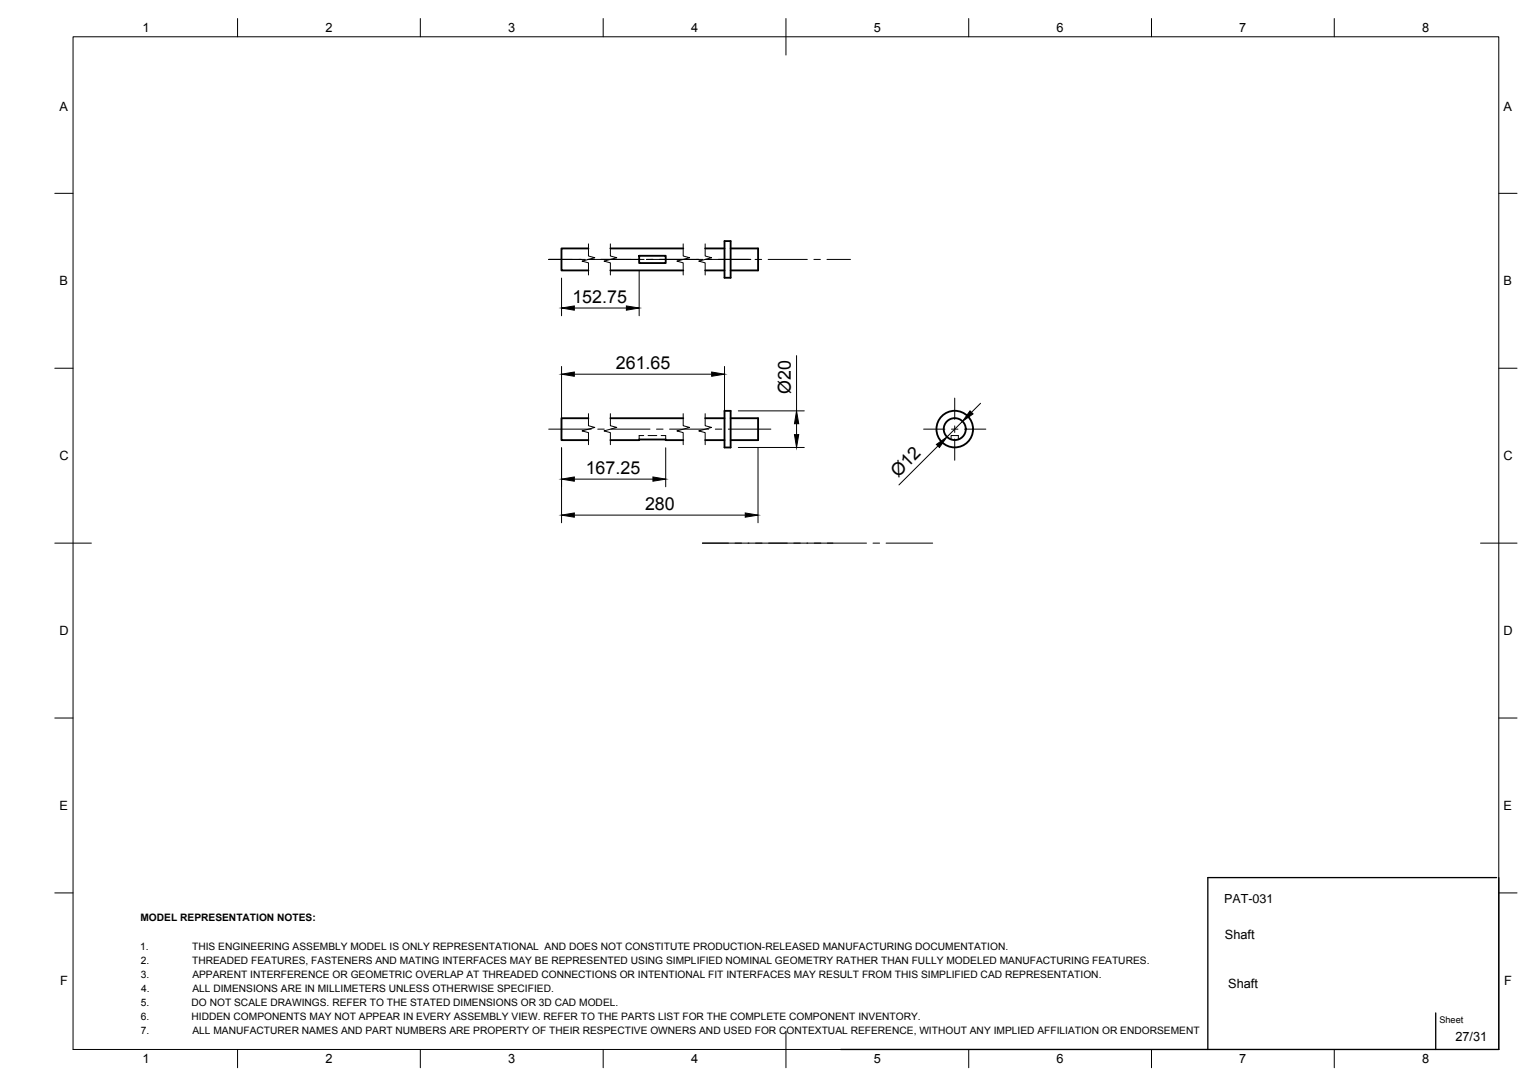
ISO-10303-21;
HEADER;
/* Generated by software containing ST-Developer
 * from STEP Tools, Inc. (www.steptools.com) 
 */

FILE_DESCRIPTION(
/* description */ ('Double-row support with tensioned shaft'),
/* implementation_level */ '2;1');

FILE_NAME(
/* name */ 'Shaft.step',
/* time_stamp */ '2026-10-27T10:50:35-07:00',
/* author */ (''),
/* organization */ (''),
/* preprocessor_version */ 'ST-DEVELOPER v20.2',
/* originating_system */ 'Autodesk Translation Framework v15.17.0.0',
/* authorisation */ '');

FILE_SCHEMA (('AUTOMOTIVE_DESIGN { 1 0 10303 214 3 1 1 }'));
ENDSEC;

DATA;
#10=MECHANICAL_DESIGN_GEOMETRIC_PRESENTATION_REPRESENTATION('',(#504),#11559);
#439=SHAPE_REPRESENTATION_RELATIONSHIP('SRR','None',#11749,#471);
#471=ADVANCED_BREP_SHAPE_REPRESENTATION('',(#534),#11551);
#504=STYLED_ITEM('',(#11967),#534);
#534=MANIFOLD_SOLID_BREP('Body1',#6352);
#653=FACE_BOUND('',#1644,.T.);
#654=FACE_BOUND('',#1646,.T.);
#655=FACE_BOUND('',#1650,.T.);
#860=PLANE('',#7233);
#861=PLANE('',#7234);
#862=PLANE('',#7236);
#863=PLANE('',#7237);
#864=PLANE('',#7238);
#865=PLANE('',#7240);
#866=PLANE('',#7243);
#867=PLANE('',#7251);
#868=PLANE('',#7252);
#1183=FACE_OUTER_BOUND('',#1638,.T.);
#1184=FACE_OUTER_BOUND('',#1639,.T.);
#1185=FACE_OUTER_BOUND('',#1640,.T.);
#1186=FACE_OUTER_BOUND('',#1641,.T.);
#1187=FACE_OUTER_BOUND('',#1642,.T.);
#1188=FACE_OUTER_BOUND('',#1643,.T.);
#1189=FACE_OUTER_BOUND('',#1645,.T.);
#1190=FACE_OUTER_BOUND('',#1647,.T.);
#1191=FACE_OUTER_BOUND('',#1648,.T.);
#1192=FACE_OUTER_BOUND('',#1649,.T.);
#1193=FACE_OUTER_BOUND('',#1651,.T.);
#1194=FACE_OUTER_BOUND('',#1652,.T.);
#1638=EDGE_LOOP('',(#5556,#5557,#5558,#5559));
#1639=EDGE_LOOP('',(#5560,#5561,#5562,#5563));
#1640=EDGE_LOOP('',(#5564,#5565,#5566,#5567));
#1641=EDGE_LOOP('',(#5568,#5569,#5570,#5571));
#1642=EDGE_LOOP('',(#5572,#5573,#5574,#5575));
#1643=EDGE_LOOP('',(#5576));
#1644=EDGE_LOOP('',(#5577));
#1645=EDGE_LOOP('',(#5578));
#1646=EDGE_LOOP('',(#5579));
#1647=EDGE_LOOP('',(#5580,#5581,#5582,#5583));
#1648=EDGE_LOOP('',(#5584,#5585,#5586,#5587));
#1649=EDGE_LOOP('',(#5588,#5589,#5590,#5591));
#1650=EDGE_LOOP('',(#5592,#5593,#5594,#5595));
#1651=EDGE_LOOP('',(#5596));
#1652=EDGE_LOOP('',(#5597));
#2169=LINE('',#11064,#2716);
#2170=LINE('',#11066,#2717);
#2171=LINE('',#11068,#2718);
#2172=LINE('',#11069,#2719);
#2173=LINE('',#11074,#2720);
#2174=LINE('',#11075,#2721);
#2175=LINE('',#11078,#2722);
#2176=LINE('',#11080,#2723);
#2177=LINE('',#11081,#2724);
#2178=LINE('',#11083,#2725);
#2179=LINE('',#11097,#2726);
#2180=LINE('',#11100,#2727);
#2181=LINE('',#11105,#2728);
#2716=VECTOR('',#8840,1.);
#2717=VECTOR('',#8841,1.);
#2718=VECTOR('',#8842,1.);
#2719=VECTOR('',#8843,1.);
#2720=VECTOR('',#8848,1.);
#2721=VECTOR('',#8849,1.);
#2722=VECTOR('',#8852,1.);
#2723=VECTOR('',#8853,1.);
#2724=VECTOR('',#8854,1.);
#2725=VECTOR('',#8857,1.);
#2726=VECTOR('',#8876,1.);
#2727=VECTOR('',#8879,0.6);
#2728=VECTOR('',#8886,0.6);
#2984=CIRCLE('',#7235,0.6);
#2985=CIRCLE('',#7239,0.6);
#2986=CIRCLE('',#7241,1.);
#2987=CIRCLE('',#7242,0.6);
#2988=CIRCLE('',#7244,1.);
#2989=CIRCLE('',#7245,0.6);
#2990=CIRCLE('',#7248,0.6);
#2991=CIRCLE('',#7250,0.6);
#3439=VERTEX_POINT('',#11062);
#3440=VERTEX_POINT('',#11063);
#3441=VERTEX_POINT('',#11065);
#3442=VERTEX_POINT('',#11067);
#3443=VERTEX_POINT('',#11071);
#3444=VERTEX_POINT('',#11073);
#3445=VERTEX_POINT('',#11077);
#3446=VERTEX_POINT('',#11079);
#3447=VERTEX_POINT('',#11087);
#3448=VERTEX_POINT('',#11089);
#3449=VERTEX_POINT('',#11092);
#3450=VERTEX_POINT('',#11094);
#3451=VERTEX_POINT('',#11099);
#3452=VERTEX_POINT('',#11103);
#4163=EDGE_CURVE('',#3439,#3440,#2169,.T.);
#4164=EDGE_CURVE('',#3439,#3441,#2170,.T.);
#4165=EDGE_CURVE('',#3442,#3441,#2171,.T.);
#4166=EDGE_CURVE('',#3442,#3440,#2172,.T.);
#4167=EDGE_CURVE('',#3440,#3443,#2984,.T.);
#4168=EDGE_CURVE('',#3444,#3442,#2173,.T.);
#4169=EDGE_CURVE('',#3443,#3444,#2174,.T.);
#4170=EDGE_CURVE('',#3443,#3445,#2175,.T.);
#4171=EDGE_CURVE('',#3444,#3446,#2176,.T.);
#4172=EDGE_CURVE('',#3446,#3445,#2177,.T.);
#4173=EDGE_CURVE('',#3441,#3446,#2178,.T.);
#4174=EDGE_CURVE('',#3445,#3439,#2985,.T.);
#4175=EDGE_CURVE('',#3447,#3447,#2986,.T.);
#4176=EDGE_CURVE('',#3448,#3448,#2987,.T.);
#4177=EDGE_CURVE('',#3449,#3449,#2988,.T.);
#4178=EDGE_CURVE('',#3450,#3450,#2989,.T.);
#4179=EDGE_CURVE('',#3447,#3449,#2179,.T.);
#4180=EDGE_CURVE('',#3450,#3451,#2180,.T.);
#4181=EDGE_CURVE('',#3451,#3451,#2990,.T.);
#4182=EDGE_CURVE('',#3452,#3452,#2991,.T.);
#4183=EDGE_CURVE('',#3452,#3448,#2181,.T.);
#5556=ORIENTED_EDGE('',*,*,#4163,.F.);
#5557=ORIENTED_EDGE('',*,*,#4164,.T.);
#5558=ORIENTED_EDGE('',*,*,#4165,.F.);
#5559=ORIENTED_EDGE('',*,*,#4166,.T.);
#5560=ORIENTED_EDGE('',*,*,#4167,.F.);
#5561=ORIENTED_EDGE('',*,*,#4166,.F.);
#5562=ORIENTED_EDGE('',*,*,#4168,.F.);
#5563=ORIENTED_EDGE('',*,*,#4169,.F.);
#5564=ORIENTED_EDGE('',*,*,#4170,.F.);
#5565=ORIENTED_EDGE('',*,*,#4169,.T.);
#5566=ORIENTED_EDGE('',*,*,#4171,.T.);
#5567=ORIENTED_EDGE('',*,*,#4172,.T.);
#5568=ORIENTED_EDGE('',*,*,#4168,.T.);
#5569=ORIENTED_EDGE('',*,*,#4165,.T.);
#5570=ORIENTED_EDGE('',*,*,#4173,.T.);
#5571=ORIENTED_EDGE('',*,*,#4171,.F.);
#5572=ORIENTED_EDGE('',*,*,#4174,.F.);
#5573=ORIENTED_EDGE('',*,*,#4172,.F.);
#5574=ORIENTED_EDGE('',*,*,#4173,.F.);
#5575=ORIENTED_EDGE('',*,*,#4164,.F.);
#5576=ORIENTED_EDGE('',*,*,#4175,.T.);
#5577=ORIENTED_EDGE('',*,*,#4176,.F.);
#5578=ORIENTED_EDGE('',*,*,#4177,.F.);
#5579=ORIENTED_EDGE('',*,*,#4178,.F.);
#5580=ORIENTED_EDGE('',*,*,#4175,.F.);
#5581=ORIENTED_EDGE('',*,*,#4179,.T.);
#5582=ORIENTED_EDGE('',*,*,#4177,.T.);
#5583=ORIENTED_EDGE('',*,*,#4179,.F.);
#5584=ORIENTED_EDGE('',*,*,#4178,.T.);
#5585=ORIENTED_EDGE('',*,*,#4180,.T.);
#5586=ORIENTED_EDGE('',*,*,#4181,.T.);
#5587=ORIENTED_EDGE('',*,*,#4180,.F.);
#5588=ORIENTED_EDGE('',*,*,#4182,.F.);
#5589=ORIENTED_EDGE('',*,*,#4183,.T.);
#5590=ORIENTED_EDGE('',*,*,#4176,.T.);
#5591=ORIENTED_EDGE('',*,*,#4183,.F.);
#5592=ORIENTED_EDGE('',*,*,#4170,.T.);
#5593=ORIENTED_EDGE('',*,*,#4174,.T.);
#5594=ORIENTED_EDGE('',*,*,#4163,.T.);
#5595=ORIENTED_EDGE('',*,*,#4167,.T.);
#5596=ORIENTED_EDGE('',*,*,#4182,.T.);
#5597=ORIENTED_EDGE('',*,*,#4181,.F.);
#5961=CYLINDRICAL_SURFACE('',#7246,1.);
#5962=CYLINDRICAL_SURFACE('',#7247,0.6);
#5963=CYLINDRICAL_SURFACE('',#7249,0.6);
#6246=ADVANCED_FACE('',(#1183),#860,.F.);
#6247=ADVANCED_FACE('',(#1184),#861,.T.);
#6248=ADVANCED_FACE('',(#1185),#862,.F.);
#6249=ADVANCED_FACE('',(#1186),#863,.F.);
#6250=ADVANCED_FACE('',(#1187),#864,.F.);
#6251=ADVANCED_FACE('',(#1188,#653),#865,.T.);
#6252=ADVANCED_FACE('',(#1189,#654),#866,.F.);
#6253=ADVANCED_FACE('',(#1190),#5961,.T.);
#6254=ADVANCED_FACE('',(#1191),#5962,.T.);
#6255=ADVANCED_FACE('',(#1192,#655),#5963,.T.);
#6256=ADVANCED_FACE('',(#1193),#867,.T.);
#6257=ADVANCED_FACE('',(#1194),#868,.F.);
#6352=CLOSED_SHELL('',(#6246,#6247,#6248,#6249,#6250,#6251,#6252,#6253,
#6254,#6255,#6256,#6257));
#7232=AXIS2_PLACEMENT_3D('',#11060,#8836,#8837);
#7233=AXIS2_PLACEMENT_3D('',#11061,#8838,#8839);
#7234=AXIS2_PLACEMENT_3D('',#11070,#8844,#8845);
#7235=AXIS2_PLACEMENT_3D('',#11072,#8846,#8847);
#7236=AXIS2_PLACEMENT_3D('',#11076,#8850,#8851);
#7237=AXIS2_PLACEMENT_3D('',#11082,#8855,#8856);
#7238=AXIS2_PLACEMENT_3D('',#11084,#8858,#8859);
#7239=AXIS2_PLACEMENT_3D('',#11085,#8860,#8861);
#7240=AXIS2_PLACEMENT_3D('',#11086,#8862,#8863);
#7241=AXIS2_PLACEMENT_3D('',#11088,#8864,#8865);
#7242=AXIS2_PLACEMENT_3D('',#11090,#8866,#8867);
#7243=AXIS2_PLACEMENT_3D('',#11091,#8868,#8869);
#7244=AXIS2_PLACEMENT_3D('',#11093,#8870,#8871);
#7245=AXIS2_PLACEMENT_3D('',#11095,#8872,#8873);
#7246=AXIS2_PLACEMENT_3D('',#11096,#8874,#8875);
#7247=AXIS2_PLACEMENT_3D('',#11098,#8877,#8878);
#7248=AXIS2_PLACEMENT_3D('',#11101,#8880,#8881);
#7249=AXIS2_PLACEMENT_3D('',#11102,#8882,#8883);
#7250=AXIS2_PLACEMENT_3D('',#11104,#8884,#8885);
#7251=AXIS2_PLACEMENT_3D('',#11106,#8887,#8888);
#7252=AXIS2_PLACEMENT_3D('',#11107,#8889,#8890);
#8836=DIRECTION('axis',(0.,0.,1.));
#8837=DIRECTION('refdir',(1.,0.,0.));
#8838=DIRECTION('center_axis',(-1.,0.,0.));
#8839=DIRECTION('ref_axis',(0.,0.,1.));
#8840=DIRECTION('',(0.,-1.,0.));
#8841=DIRECTION('',(0.,0.,1.));
#8842=DIRECTION('',(0.,1.,0.));
#8843=DIRECTION('',(0.,0.,-1.));
#8844=DIRECTION('center_axis',(0.,1.,0.));
#8845=DIRECTION('ref_axis',(1.,0.,0.));
#8846=DIRECTION('center_axis',(0.,-1.,0.));
#8847=DIRECTION('ref_axis',(1.,0.,0.));
#8848=DIRECTION('',(-1.,0.,0.));
#8849=DIRECTION('',(0.,0.,1.));
#8850=DIRECTION('center_axis',(1.,0.,0.));
#8851=DIRECTION('ref_axis',(0.,0.,-1.));
#8852=DIRECTION('',(0.,1.,0.));
#8853=DIRECTION('',(0.,1.,0.));
#8854=DIRECTION('',(0.,0.,-1.));
#8855=DIRECTION('center_axis',(0.,0.,1.));
#8856=DIRECTION('ref_axis',(1.,0.,0.));
#8857=DIRECTION('',(1.,0.,0.));
#8858=DIRECTION('center_axis',(0.,1.,0.));
#8859=DIRECTION('ref_axis',(0.,0.,1.));
#8860=DIRECTION('center_axis',(0.,1.,0.));
#8861=DIRECTION('ref_axis',(1.,0.,0.));
#8862=DIRECTION('center_axis',(0.,1.,0.));
#8863=DIRECTION('ref_axis',(1.,0.,0.));
#8864=DIRECTION('center_axis',(0.,1.,0.));
#8865=DIRECTION('ref_axis',(1.,0.,0.));
#8866=DIRECTION('center_axis',(0.,1.,0.));
#8867=DIRECTION('ref_axis',(1.,0.,0.));
#8868=DIRECTION('center_axis',(0.,1.,0.));
#8869=DIRECTION('ref_axis',(1.,0.,0.));
#8870=DIRECTION('center_axis',(0.,1.,0.));
#8871=DIRECTION('ref_axis',(1.,0.,0.));
#8872=DIRECTION('center_axis',(0.,-1.,0.));
#8873=DIRECTION('ref_axis',(1.,0.,0.));
#8874=DIRECTION('center_axis',(0.,1.,0.));
#8875=DIRECTION('ref_axis',(1.,0.,0.));
#8876=DIRECTION('',(0.,-1.,0.));
#8877=DIRECTION('center_axis',(0.,1.,0.));
#8878=DIRECTION('ref_axis',(1.,0.,0.));
#8879=DIRECTION('',(0.,-1.,0.));
#8880=DIRECTION('center_axis',(0.,1.,0.));
#8881=DIRECTION('ref_axis',(1.,0.,0.));
#8882=DIRECTION('center_axis',(0.,1.,0.));
#8883=DIRECTION('ref_axis',(1.,0.,0.));
#8884=DIRECTION('center_axis',(0.,1.,0.));
#8885=DIRECTION('ref_axis',(1.,0.,0.));
#8886=DIRECTION('',(0.,-1.,0.));
#8887=DIRECTION('center_axis',(0.,1.,0.));
#8888=DIRECTION('ref_axis',(1.,0.,0.));
#8889=DIRECTION('center_axis',(0.,1.,0.));
#8890=DIRECTION('ref_axis',(1.,0.,0.));
#11060=CARTESIAN_POINT('',(0.,0.,0.));
#11061=CARTESIAN_POINT('Origin',(-0.2,7.775,9.3));
#11062=CARTESIAN_POINT('',(-0.2,9.225,9.43431457505076));
#11063=CARTESIAN_POINT('',(-0.2,7.775,9.43431457505076));
#11064=CARTESIAN_POINT('',(-0.2,-3.5,9.43431457505076));
#11065=CARTESIAN_POINT('',(-0.2,9.225,9.65));
#11066=CARTESIAN_POINT('',(-0.2,9.225,9.65));
#11067=CARTESIAN_POINT('',(-0.2,7.775,9.65));
#11068=CARTESIAN_POINT('',(-0.2,7.775,9.65));
#11069=CARTESIAN_POINT('',(-0.2,7.775,9.65));
#11070=CARTESIAN_POINT('Origin',(0.,7.775,9.475));
#11071=CARTESIAN_POINT('',(0.2,7.775,9.43431457505076));
#11072=CARTESIAN_POINT('Origin',(0.,7.775,10.));
#11073=CARTESIAN_POINT('',(0.2,7.775,9.65));
#11074=CARTESIAN_POINT('',(0.2,7.775,9.65));
#11075=CARTESIAN_POINT('',(0.2,7.775,9.3));
#11076=CARTESIAN_POINT('Origin',(0.2,7.775,9.65));
#11077=CARTESIAN_POINT('',(0.2,9.225,9.43431457505076));
#11078=CARTESIAN_POINT('',(0.2,-3.5,9.43431457505076));
#11079=CARTESIAN_POINT('',(0.2,9.225,9.65));
#11080=CARTESIAN_POINT('',(0.2,7.775,9.65));
#11081=CARTESIAN_POINT('',(0.2,9.225,9.3));
#11082=CARTESIAN_POINT('Origin',(-0.2,7.775,9.65));
#11083=CARTESIAN_POINT('',(0.2,9.225,9.65));
#11084=CARTESIAN_POINT('Origin',(0.,9.225,9.475));
#11085=CARTESIAN_POINT('Origin',(0.,9.225,10.));
#11086=CARTESIAN_POINT('Origin',(0.,-1.665,10.));
#11087=CARTESIAN_POINT('',(-1.,-1.665,10.));
#11088=CARTESIAN_POINT('Origin',(0.,-1.665,10.));
#11089=CARTESIAN_POINT('',(-0.6,-1.665,10.));
#11090=CARTESIAN_POINT('Origin',(0.,-1.665,10.));
#11091=CARTESIAN_POINT('Origin',(0.,-2.,10.));
#11092=CARTESIAN_POINT('',(-1.,-2.,10.));
#11093=CARTESIAN_POINT('Origin',(0.,-2.,10.));
#11094=CARTESIAN_POINT('',(-0.6,-2.,10.));
#11095=CARTESIAN_POINT('Origin',(0.,-2.,10.));
#11096=CARTESIAN_POINT('Origin',(0.,-2.,10.));
#11097=CARTESIAN_POINT('',(-1.,-2.,10.));
#11098=CARTESIAN_POINT('Origin',(0.,-3.5,10.));
#11099=CARTESIAN_POINT('',(-0.6,-3.5,10.));
#11100=CARTESIAN_POINT('',(-0.6,-3.5,10.));
#11101=CARTESIAN_POINT('Origin',(0.,-3.5,10.));
#11102=CARTESIAN_POINT('Origin',(0.,-3.5,10.));
#11103=CARTESIAN_POINT('',(-0.6,24.5,10.));
#11104=CARTESIAN_POINT('Origin',(0.,24.5,10.));
#11105=CARTESIAN_POINT('',(-0.6,-3.5,10.));
#11106=CARTESIAN_POINT('Origin',(0.,24.5,10.));
#11107=CARTESIAN_POINT('Origin',(0.,-3.5,10.));
#11514=UNCERTAINTY_MEASURE_WITH_UNIT(LENGTH_MEASURE(0.001),#11560,
'DISTANCE_ACCURACY_VALUE',
'Maximum model space distance between geometric entities at asserted c
onnectivities');
#11522=UNCERTAINTY_MEASURE_WITH_UNIT(LENGTH_MEASURE(0.001),#11560,
'DISTANCE_ACCURACY_VALUE',
'Maximum model space distance between geometric entities at asserted c
onnectivities');
#11551=(
GEOMETRIC_REPRESENTATION_CONTEXT(3)
GLOBAL_UNCERTAINTY_ASSIGNED_CONTEXT((#11514))
GLOBAL_UNIT_ASSIGNED_CONTEXT((#11560,#11562,#11563))
REPRESENTATION_CONTEXT('','3D')
);
#11559=(
GEOMETRIC_REPRESENTATION_CONTEXT(3)
GLOBAL_UNCERTAINTY_ASSIGNED_CONTEXT((#11522))
GLOBAL_UNIT_ASSIGNED_CONTEXT((#11560,#11562,#11563))
REPRESENTATION_CONTEXT('','3D')
);
#11560=(
LENGTH_UNIT()
NAMED_UNIT(*)
SI_UNIT(.CENTI.,.METRE.)
);
#11562=(
NAMED_UNIT(*)
PLANE_ANGLE_UNIT()
SI_UNIT($,.RADIAN.)
);
#11563=(
NAMED_UNIT(*)
SI_UNIT($,.STERADIAN.)
SOLID_ANGLE_UNIT()
);
#11592=SHAPE_DEFINITION_REPRESENTATION(#11703,#11749);
#11703=PRODUCT_DEFINITION_SHAPE('',$,#11786);
#11749=SHAPE_REPRESENTATION('',(#7232),#11551);
#11757=PRODUCT_DEFINITION_CONTEXT('part definition',#11867,'design');
#11786=PRODUCT_DEFINITION('Shaft','Shaft',#11822,#11757);
#11822=PRODUCT_DEFINITION_FORMATION('',$,#11897);
#11867=APPLICATION_CONTEXT(
'Core Data for Automotive Mechanical Design Process');
#11868=PRODUCT_CONTEXT('part definition',#11867,'mechanical');
#11897=PRODUCT('Shaft','Shaft','Shaft',(#11868));
#11961=COLOUR_RGB('Grey',0.48,0.52,0.57);
#11962=FILL_AREA_STYLE_COLOUR('',#11961);
#11963=FILL_AREA_STYLE('',(#11962));
#11964=SURFACE_STYLE_FILL_AREA(#11963);
#11965=SURFACE_SIDE_STYLE('',(#11964));
#11966=SURFACE_STYLE_USAGE(.BOTH.,#11965);
#11967=PRESENTATION_STYLE_ASSIGNMENT((#11966));
ENDSEC;
END-ISO-10303-21;
